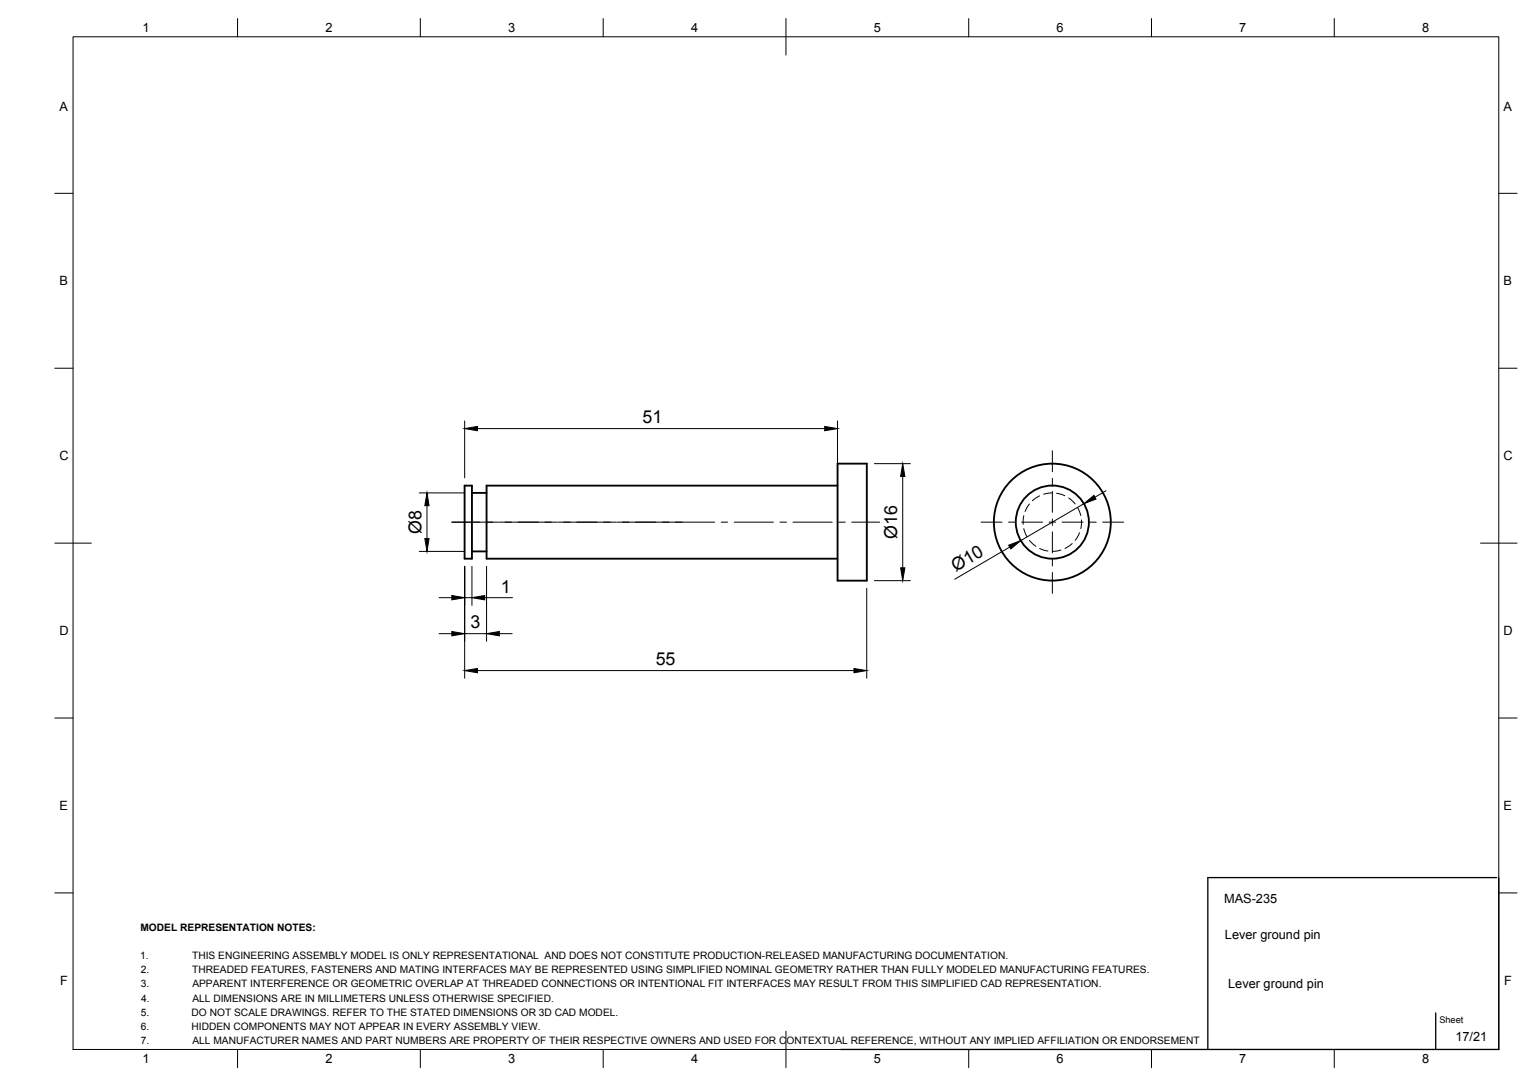
ISO-10303-21;
HEADER;
/* Generated by software containing ST-Developer
 * from STEP Tools, Inc. (www.steptools.com) 
 */

FILE_DESCRIPTION(
/* description */ ('Independent Whitworth quick-return mechanism. Crank radius40, ground-
center spacing80, lever180, connecting rod160, output guide X200. Nomi
nal stroke180 and long/short phase ratio2. Retained guide rods, replac
eable bearing sleeves and captured sliding shoe. No load or production
 rating assigned.'),
/* implementation_level */ '2;1');

FILE_NAME(
/* name */ 'Lever ground pin.step',
/* time_stamp */ '2026-11-09T18:22:56-08:00',
/* author */ (''),
/* organization */ (''),
/* preprocessor_version */ 'ST-DEVELOPER v20.2',
/* originating_system */ 'Autodesk Translation Framework v15.17.0.0',
/* authorisation */ '');

FILE_SCHEMA (('AUTOMOTIVE_DESIGN { 1 0 10303 214 3 1 1 }'));
ENDSEC;

DATA;
#10=MECHANICAL_DESIGN_GEOMETRIC_PRESENTATION_REPRESENTATION('',(#231),#4388);
#191=SHAPE_REPRESENTATION_RELATIONSHIP('SRR','None',#4490,#211);
#211=ADVANCED_BREP_SHAPE_REPRESENTATION('',(#251),#4380);
#231=STYLED_ITEM('',(#4595),#251);
#251=MANIFOLD_SOLID_BREP('Body1',#2336);
#299=FACE_BOUND('',#683,.T.);
#300=FACE_BOUND('',#685,.T.);
#301=FACE_BOUND('',#688,.T.);
#373=PLANE('',#2741);
#374=PLANE('',#2743);
#375=PLANE('',#2747);
#376=PLANE('',#2752);
#377=PLANE('',#2754);
#494=FACE_OUTER_BOUND('',#681,.T.);
#495=FACE_OUTER_BOUND('',#682,.T.);
#496=FACE_OUTER_BOUND('',#684,.T.);
#497=FACE_OUTER_BOUND('',#686,.T.);
#498=FACE_OUTER_BOUND('',#687,.T.);
#499=FACE_OUTER_BOUND('',#689,.T.);
#500=FACE_OUTER_BOUND('',#690,.T.);
#501=FACE_OUTER_BOUND('',#691,.T.);
#502=FACE_OUTER_BOUND('',#692,.T.);
#681=EDGE_LOOP('',(#1948,#1949,#1950,#1951));
#682=EDGE_LOOP('',(#1952));
#683=EDGE_LOOP('',(#1953));
#684=EDGE_LOOP('',(#1954));
#685=EDGE_LOOP('',(#1955));
#686=EDGE_LOOP('',(#1956,#1957,#1958,#1959));
#687=EDGE_LOOP('',(#1960));
#688=EDGE_LOOP('',(#1961));
#689=EDGE_LOOP('',(#1962,#1963,#1964,#1965));
#690=EDGE_LOOP('',(#1966));
#691=EDGE_LOOP('',(#1967,#1968,#1969,#1970));
#692=EDGE_LOOP('',(#1971));
#866=LINE('',#4102,#1005);
#867=LINE('',#4113,#1006);
#868=LINE('',#4121,#1007);
#869=LINE('',#4125,#1008);
#1005=VECTOR('',#3354,4.);
#1006=VECTOR('',#3369,5.);
#1007=VECTOR('',#3378,8.);
#1008=VECTOR('',#3385,5.);
#1107=CIRCLE('',#2739,4.);
#1108=CIRCLE('',#2740,4.);
#1109=CIRCLE('',#2742,5.);
#1110=CIRCLE('',#2744,5.);
#1111=CIRCLE('',#2746,5.);
#1112=CIRCLE('',#2748,8.);
#1113=CIRCLE('',#2749,5.);
#1114=CIRCLE('',#2751,8.);
#1277=VERTEX_POINT('',#4099);
#1278=VERTEX_POINT('',#4101);
#1279=VERTEX_POINT('',#4105);
#1280=VERTEX_POINT('',#4108);
#1281=VERTEX_POINT('',#4111);
#1282=VERTEX_POINT('',#4115);
#1283=VERTEX_POINT('',#4117);
#1284=VERTEX_POINT('',#4120);
#1510=EDGE_CURVE('',#1277,#1277,#1107,.T.);
#1511=EDGE_CURVE('',#1277,#1278,#866,.T.);
#1512=EDGE_CURVE('',#1278,#1278,#1108,.T.);
#1513=EDGE_CURVE('',#1279,#1279,#1109,.T.);
#1514=EDGE_CURVE('',#1280,#1280,#1110,.T.);
#1515=EDGE_CURVE('',#1281,#1281,#1111,.T.);
#1516=EDGE_CURVE('',#1281,#1280,#867,.T.);
#1517=EDGE_CURVE('',#1282,#1282,#1112,.T.);
#1518=EDGE_CURVE('',#1283,#1283,#1113,.T.);
#1519=EDGE_CURVE('',#1282,#1284,#868,.T.);
#1520=EDGE_CURVE('',#1284,#1284,#1114,.T.);
#1521=EDGE_CURVE('',#1279,#1283,#869,.T.);
#1948=ORIENTED_EDGE('',*,*,#1510,.T.);
#1949=ORIENTED_EDGE('',*,*,#1511,.T.);
#1950=ORIENTED_EDGE('',*,*,#1512,.F.);
#1951=ORIENTED_EDGE('',*,*,#1511,.F.);
#1952=ORIENTED_EDGE('',*,*,#1513,.F.);
#1953=ORIENTED_EDGE('',*,*,#1510,.F.);
#1954=ORIENTED_EDGE('',*,*,#1514,.F.);
#1955=ORIENTED_EDGE('',*,*,#1512,.T.);
#1956=ORIENTED_EDGE('',*,*,#1515,.F.);
#1957=ORIENTED_EDGE('',*,*,#1516,.T.);
#1958=ORIENTED_EDGE('',*,*,#1514,.T.);
#1959=ORIENTED_EDGE('',*,*,#1516,.F.);
#1960=ORIENTED_EDGE('',*,*,#1517,.T.);
#1961=ORIENTED_EDGE('',*,*,#1518,.F.);
#1962=ORIENTED_EDGE('',*,*,#1517,.F.);
#1963=ORIENTED_EDGE('',*,*,#1519,.T.);
#1964=ORIENTED_EDGE('',*,*,#1520,.T.);
#1965=ORIENTED_EDGE('',*,*,#1519,.F.);
#1966=ORIENTED_EDGE('',*,*,#1520,.F.);
#1967=ORIENTED_EDGE('',*,*,#1513,.T.);
#1968=ORIENTED_EDGE('',*,*,#1521,.T.);
#1969=ORIENTED_EDGE('',*,*,#1518,.T.);
#1970=ORIENTED_EDGE('',*,*,#1521,.F.);
#1971=ORIENTED_EDGE('',*,*,#1515,.T.);
#2151=CYLINDRICAL_SURFACE('',#2738,4.);
#2152=CYLINDRICAL_SURFACE('',#2745,5.);
#2153=CYLINDRICAL_SURFACE('',#2750,8.);
#2154=CYLINDRICAL_SURFACE('',#2753,5.);
#2266=ADVANCED_FACE('',(#494),#2151,.T.);
#2267=ADVANCED_FACE('',(#495,#299),#373,.F.);
#2268=ADVANCED_FACE('',(#496,#300),#374,.F.);
#2269=ADVANCED_FACE('',(#497),#2152,.T.);
#2270=ADVANCED_FACE('',(#498,#301),#375,.T.);
#2271=ADVANCED_FACE('',(#499),#2153,.T.);
#2272=ADVANCED_FACE('',(#500),#376,.F.);
#2273=ADVANCED_FACE('',(#501),#2154,.T.);
#2274=ADVANCED_FACE('',(#502),#377,.T.);
#2336=CLOSED_SHELL('',(#2266,#2267,#2268,#2269,#2270,#2271,#2272,#2273,
#2274));
#2737=AXIS2_PLACEMENT_3D('',#4097,#3348,#3349);
#2738=AXIS2_PLACEMENT_3D('',#4098,#3350,#3351);
#2739=AXIS2_PLACEMENT_3D('',#4100,#3352,#3353);
#2740=AXIS2_PLACEMENT_3D('',#4103,#3355,#3356);
#2741=AXIS2_PLACEMENT_3D('',#4104,#3357,#3358);
#2742=AXIS2_PLACEMENT_3D('',#4106,#3359,#3360);
#2743=AXIS2_PLACEMENT_3D('',#4107,#3361,#3362);
#2744=AXIS2_PLACEMENT_3D('',#4109,#3363,#3364);
#2745=AXIS2_PLACEMENT_3D('',#4110,#3365,#3366);
#2746=AXIS2_PLACEMENT_3D('',#4112,#3367,#3368);
#2747=AXIS2_PLACEMENT_3D('',#4114,#3370,#3371);
#2748=AXIS2_PLACEMENT_3D('',#4116,#3372,#3373);
#2749=AXIS2_PLACEMENT_3D('',#4118,#3374,#3375);
#2750=AXIS2_PLACEMENT_3D('',#4119,#3376,#3377);
#2751=AXIS2_PLACEMENT_3D('',#4122,#3379,#3380);
#2752=AXIS2_PLACEMENT_3D('',#4123,#3381,#3382);
#2753=AXIS2_PLACEMENT_3D('',#4124,#3383,#3384);
#2754=AXIS2_PLACEMENT_3D('',#4126,#3386,#3387);
#3348=DIRECTION('axis',(0.,0.,1.));
#3349=DIRECTION('refdir',(1.,0.,0.));
#3350=DIRECTION('center_axis',(0.,0.,1.));
#3351=DIRECTION('ref_axis',(1.,0.,0.));
#3352=DIRECTION('center_axis',(0.,0.,1.));
#3353=DIRECTION('ref_axis',(1.,0.,0.));
#3354=DIRECTION('',(0.,0.,1.));
#3355=DIRECTION('center_axis',(0.,0.,1.));
#3356=DIRECTION('ref_axis',(1.,0.,0.));
#3357=DIRECTION('center_axis',(0.,0.,-1.));
#3358=DIRECTION('ref_axis',(-1.,0.,0.));
#3359=DIRECTION('center_axis',(0.,0.,-1.));
#3360=DIRECTION('ref_axis',(1.,0.,0.));
#3361=DIRECTION('center_axis',(0.,0.,1.));
#3362=DIRECTION('ref_axis',(1.,0.,0.));
#3363=DIRECTION('center_axis',(0.,0.,1.));
#3364=DIRECTION('ref_axis',(1.,0.,0.));
#3365=DIRECTION('center_axis',(0.,0.,1.));
#3366=DIRECTION('ref_axis',(1.,0.,0.));
#3367=DIRECTION('center_axis',(0.,0.,1.));
#3368=DIRECTION('ref_axis',(1.,0.,0.));
#3369=DIRECTION('',(0.,0.,-1.));
#3370=DIRECTION('center_axis',(0.,0.,1.));
#3371=DIRECTION('ref_axis',(1.,0.,0.));
#3372=DIRECTION('center_axis',(0.,0.,1.));
#3373=DIRECTION('ref_axis',(1.,0.,0.));
#3374=DIRECTION('center_axis',(0.,0.,1.));
#3375=DIRECTION('ref_axis',(1.,0.,0.));
#3376=DIRECTION('center_axis',(0.,0.,1.));
#3377=DIRECTION('ref_axis',(1.,0.,0.));
#3378=DIRECTION('',(0.,0.,-1.));
#3379=DIRECTION('center_axis',(0.,0.,1.));
#3380=DIRECTION('ref_axis',(1.,0.,0.));
#3381=DIRECTION('center_axis',(0.,0.,1.));
#3382=DIRECTION('ref_axis',(1.,0.,0.));
#3383=DIRECTION('center_axis',(0.,0.,1.));
#3384=DIRECTION('ref_axis',(1.,0.,0.));
#3385=DIRECTION('',(0.,0.,-1.));
#3386=DIRECTION('center_axis',(0.,0.,1.));
#3387=DIRECTION('ref_axis',(1.,0.,0.));
#4097=CARTESIAN_POINT('',(0.,0.,0.));
#4098=CARTESIAN_POINT('Origin',(0.,0.,49.));
#4099=CARTESIAN_POINT('',(-4.,-4.89858719658941E-16,48.));
#4100=CARTESIAN_POINT('Origin',(0.,0.,48.));
#4101=CARTESIAN_POINT('',(-4.,-4.89858719658941E-16,50.));
#4102=CARTESIAN_POINT('',(-4.,-4.89858719658941E-16,49.));
#4103=CARTESIAN_POINT('Origin',(0.,0.,50.));
#4104=CARTESIAN_POINT('Origin',(8.,0.,48.));
#4105=CARTESIAN_POINT('',(-5.,6.12323399573677E-16,48.));
#4106=CARTESIAN_POINT('Origin',(0.,0.,48.));
#4107=CARTESIAN_POINT('Origin',(4.,0.,50.));
#4108=CARTESIAN_POINT('',(-5.,-6.12323399573677E-16,50.));
#4109=CARTESIAN_POINT('Origin',(0.,0.,50.));
#4110=CARTESIAN_POINT('Origin',(0.,0.,0.));
#4111=CARTESIAN_POINT('',(-5.,-6.12323399573677E-16,51.));
#4112=CARTESIAN_POINT('Origin',(0.,0.,51.));
#4113=CARTESIAN_POINT('',(-5.,-6.12323399573677E-16,0.));
#4114=CARTESIAN_POINT('Origin',(0.,0.,0.));
#4115=CARTESIAN_POINT('',(-8.,-9.79717439317883E-16,0.));
#4116=CARTESIAN_POINT('Origin',(0.,0.,0.));
#4117=CARTESIAN_POINT('',(-5.,-6.12323399573677E-16,0.));
#4118=CARTESIAN_POINT('Origin',(0.,0.,0.));
#4119=CARTESIAN_POINT('Origin',(0.,0.,-4.));
#4120=CARTESIAN_POINT('',(-8.,-9.79717439317883E-16,-4.));
#4121=CARTESIAN_POINT('',(-8.,-9.79717439317883E-16,-4.));
#4122=CARTESIAN_POINT('Origin',(0.,0.,-4.));
#4123=CARTESIAN_POINT('Origin',(0.,0.,-4.));
#4124=CARTESIAN_POINT('Origin',(0.,0.,0.));
#4125=CARTESIAN_POINT('',(-5.,-6.12323399573677E-16,0.));
#4126=CARTESIAN_POINT('Origin',(0.,0.,51.));
#4358=UNCERTAINTY_MEASURE_WITH_UNIT(LENGTH_MEASURE(0.01),#4389,
'DISTANCE_ACCURACY_VALUE',
'Maximum model space distance between geometric entities at asserted c
onnectivities');
#4366=UNCERTAINTY_MEASURE_WITH_UNIT(LENGTH_MEASURE(0.01),#4389,
'DISTANCE_ACCURACY_VALUE',
'Maximum model space distance between geometric entities at asserted c
onnectivities');
#4380=(
GEOMETRIC_REPRESENTATION_CONTEXT(3)
GLOBAL_UNCERTAINTY_ASSIGNED_CONTEXT((#4358))
GLOBAL_UNIT_ASSIGNED_CONTEXT((#4389,#4391,#4392))
REPRESENTATION_CONTEXT('','3D')
);
#4388=(
GEOMETRIC_REPRESENTATION_CONTEXT(3)
GLOBAL_UNCERTAINTY_ASSIGNED_CONTEXT((#4366))
GLOBAL_UNIT_ASSIGNED_CONTEXT((#4389,#4391,#4392))
REPRESENTATION_CONTEXT('','3D')
);
#4389=(
LENGTH_UNIT()
NAMED_UNIT(*)
SI_UNIT(.MILLI.,.METRE.)
);
#4391=(
NAMED_UNIT(*)
PLANE_ANGLE_UNIT()
SI_UNIT($,.RADIAN.)
);
#4392=(
NAMED_UNIT(*)
SI_UNIT($,.STERADIAN.)
SOLID_ANGLE_UNIT()
);
#4406=SHAPE_DEFINITION_REPRESENTATION(#4427,#4490);
#4427=PRODUCT_DEFINITION_SHAPE('',$,#4512);
#4490=SHAPE_REPRESENTATION('',(#2737),#4380);
#4498=PRODUCT_DEFINITION_CONTEXT('part definition',#4563,'design');
#4512=PRODUCT_DEFINITION('Lever ground pin','Lever ground pin',#4533,#4498);
#4533=PRODUCT_DEFINITION_FORMATION('',$,#4578);
#4563=APPLICATION_CONTEXT(
'Core Data for Automotive Mechanical Design Process');
#4564=PRODUCT_CONTEXT('part definition',#4563,'mechanical');
#4578=PRODUCT('Lever ground pin','Lever ground pin',$,(#4564));
#4595=PRESENTATION_STYLE_ASSIGNMENT((#4609));
#4609=SURFACE_STYLE_USAGE(.BOTH.,#4623);
#4623=SURFACE_SIDE_STYLE('',(#4637));
#4637=SURFACE_STYLE_FILL_AREA(#4651);
#4651=FILL_AREA_STYLE('Pivot gray',(#4665));
#4665=FILL_AREA_STYLE_COLOUR('Pivot gray',#4679);
#4679=COLOUR_RGB('Pivot gray',0.407843137254902,0.447058823529412,0.498039215686275);
ENDSEC;
END-ISO-10303-21;
